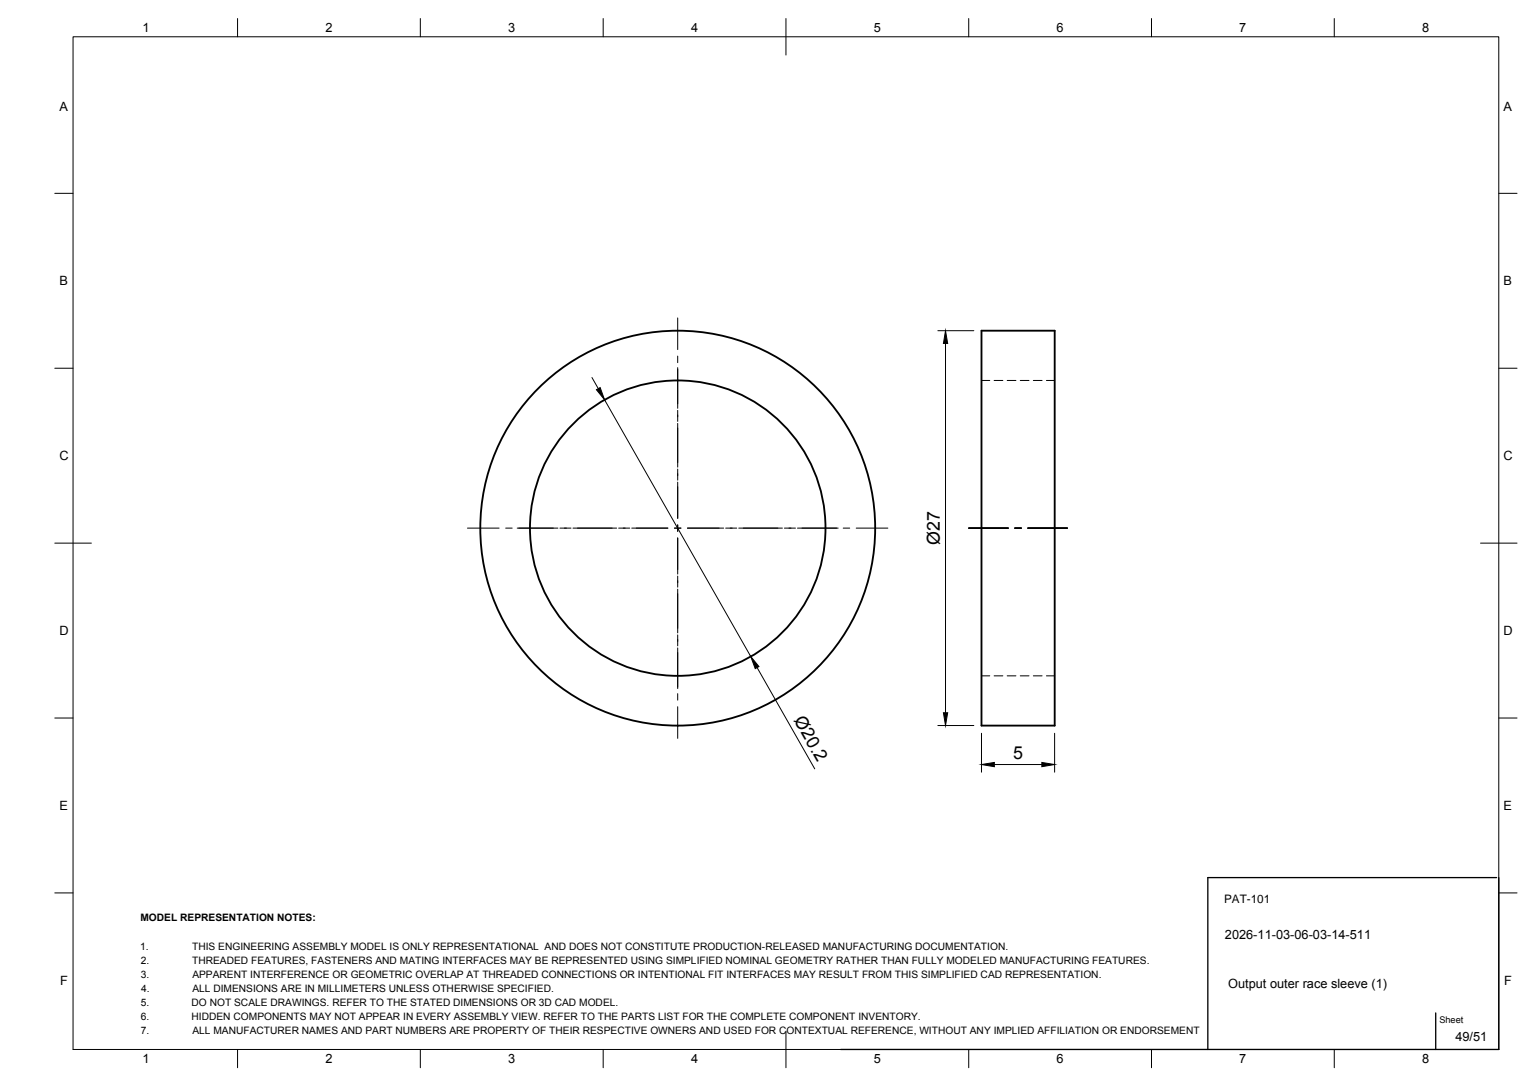
ISO-10303-21;
HEADER;
/* Generated by software containing ST-Developer
 * from STEP Tools, Inc. (www.steptools.com) 
 */

FILE_DESCRIPTION(
/* description */ ('Spur gear reduction stage 2-1 on bearing plates'),
/* implementation_level */ '2;1');

FILE_NAME(
/* name */ 'Output outer race sleeve (1).step',
/* time_stamp */ '2026-10-28T03:22:07-07:00',
/* author */ (''),
/* organization */ (''),
/* preprocessor_version */ 'ST-DEVELOPER v20.2',
/* originating_system */ 'Autodesk Translation Framework v15.17.0.0',
/* authorisation */ '');

FILE_SCHEMA (('AUTOMOTIVE_DESIGN { 1 0 10303 214 3 1 1 }'));
ENDSEC;

DATA;
#10=MECHANICAL_DESIGN_GEOMETRIC_PRESENTATION_REPRESENTATION('',(#1001),#53909);
#900=SHAPE_REPRESENTATION_RELATIONSHIP('SRR','None',#54131,#943);
#943=ADVANCED_BREP_SHAPE_REPRESENTATION('',(#1056),#53905);
#1001=STYLED_ITEM('',(#54397),#1056);
#1056=MANIFOLD_SOLID_BREP('Body1',#11328);
#1232=FACE_BOUND('',#2780,.T.);
#1233=FACE_BOUND('',#2782,.T.);
#1436=PLANE('',#12754);
#1437=PLANE('',#12755);
#1957=FACE_OUTER_BOUND('',#2777,.T.);
#1958=FACE_OUTER_BOUND('',#2778,.T.);
#1959=FACE_OUTER_BOUND('',#2779,.T.);
#1960=FACE_OUTER_BOUND('',#2781,.T.);
#2777=EDGE_LOOP('',(#9320,#9321,#9322,#9323));
#2778=EDGE_LOOP('',(#9324,#9325,#9326,#9327));
#2779=EDGE_LOOP('',(#9328));
#2780=EDGE_LOOP('',(#9329));
#2781=EDGE_LOOP('',(#9330));
#2782=EDGE_LOOP('',(#9331));
#3400=LINE('',#30116,#4041);
#3401=LINE('',#30122,#4042);
#4041=VECTOR('',#15293,1.01);
#4042=VECTOR('',#15300,1.35);
#4692=CIRCLE('',#12749,1.01);
#4693=CIRCLE('',#12750,1.01);
#4694=CIRCLE('',#12752,1.35);
#4695=CIRCLE('',#12753,1.35);
#5452=VERTEX_POINT('',#30113);
#5453=VERTEX_POINT('',#30115);
#5454=VERTEX_POINT('',#30119);
#5455=VERTEX_POINT('',#30121);
#6802=EDGE_CURVE('',#5452,#5452,#4692,.T.);
#6803=EDGE_CURVE('',#5452,#5453,#3400,.T.);
#6804=EDGE_CURVE('',#5453,#5453,#4693,.T.);
#6805=EDGE_CURVE('',#5454,#5454,#4694,.T.);
#6806=EDGE_CURVE('',#5454,#5455,#3401,.T.);
#6807=EDGE_CURVE('',#5455,#5455,#4695,.T.);
#9320=ORIENTED_EDGE('',*,*,#6802,.F.);
#9321=ORIENTED_EDGE('',*,*,#6803,.T.);
#9322=ORIENTED_EDGE('',*,*,#6804,.T.);
#9323=ORIENTED_EDGE('',*,*,#6803,.F.);
#9324=ORIENTED_EDGE('',*,*,#6805,.F.);
#9325=ORIENTED_EDGE('',*,*,#6806,.T.);
#9326=ORIENTED_EDGE('',*,*,#6807,.T.);
#9327=ORIENTED_EDGE('',*,*,#6806,.F.);
#9328=ORIENTED_EDGE('',*,*,#6805,.T.);
#9329=ORIENTED_EDGE('',*,*,#6802,.T.);
#9330=ORIENTED_EDGE('',*,*,#6807,.F.);
#9331=ORIENTED_EDGE('',*,*,#6804,.F.);
#10578=CYLINDRICAL_SURFACE('',#12748,1.01);
#10579=CYLINDRICAL_SURFACE('',#12751,1.35);
#11077=ADVANCED_FACE('',(#1957),#10578,.F.);
#11078=ADVANCED_FACE('',(#1958),#10579,.T.);
#11079=ADVANCED_FACE('',(#1959,#1232),#1436,.T.);
#11080=ADVANCED_FACE('',(#1960,#1233),#1437,.F.);
#11328=CLOSED_SHELL('',(#11077,#11078,#11079,#11080));
#12747=AXIS2_PLACEMENT_3D('',#30111,#15287,#15288);
#12748=AXIS2_PLACEMENT_3D('',#30112,#15289,#15290);
#12749=AXIS2_PLACEMENT_3D('',#30114,#15291,#15292);
#12750=AXIS2_PLACEMENT_3D('',#30117,#15294,#15295);
#12751=AXIS2_PLACEMENT_3D('',#30118,#15296,#15297);
#12752=AXIS2_PLACEMENT_3D('',#30120,#15298,#15299);
#12753=AXIS2_PLACEMENT_3D('',#30123,#15301,#15302);
#12754=AXIS2_PLACEMENT_3D('',#30124,#15303,#15304);
#12755=AXIS2_PLACEMENT_3D('',#30125,#15305,#15306);
#15287=DIRECTION('axis',(0.,0.,1.));
#15288=DIRECTION('refdir',(1.,0.,0.));
#15289=DIRECTION('center_axis',(0.,1.,0.));
#15290=DIRECTION('ref_axis',(1.,0.,0.));
#15291=DIRECTION('center_axis',(0.,-1.,0.));
#15292=DIRECTION('ref_axis',(1.,0.,0.));
#15293=DIRECTION('',(0.,-1.,0.));
#15294=DIRECTION('center_axis',(0.,-1.,0.));
#15295=DIRECTION('ref_axis',(1.,0.,0.));
#15296=DIRECTION('center_axis',(0.,1.,0.));
#15297=DIRECTION('ref_axis',(1.,0.,0.));
#15298=DIRECTION('center_axis',(0.,1.,0.));
#15299=DIRECTION('ref_axis',(1.,0.,0.));
#15300=DIRECTION('',(0.,-1.,0.));
#15301=DIRECTION('center_axis',(0.,1.,0.));
#15302=DIRECTION('ref_axis',(1.,0.,0.));
#15303=DIRECTION('center_axis',(0.,1.,0.));
#15304=DIRECTION('ref_axis',(1.,0.,0.));
#15305=DIRECTION('center_axis',(0.,1.,0.));
#15306=DIRECTION('ref_axis',(1.,0.,0.));
#30111=CARTESIAN_POINT('',(0.,0.,0.));
#30112=CARTESIAN_POINT('Origin',(0.,4.2,0.));
#30113=CARTESIAN_POINT('',(-1.01,4.7,1.23689326713883E-16));
#30114=CARTESIAN_POINT('Origin',(0.,4.7,0.));
#30115=CARTESIAN_POINT('',(-1.01,4.2,1.23689326713883E-16));
#30116=CARTESIAN_POINT('',(-1.01,4.2,1.23689326713883E-16));
#30117=CARTESIAN_POINT('Origin',(0.,4.2,0.));
#30118=CARTESIAN_POINT('Origin',(0.,4.2,0.));
#30119=CARTESIAN_POINT('',(-1.35,4.7,1.65327317884893E-16));
#30120=CARTESIAN_POINT('Origin',(0.,4.7,0.));
#30121=CARTESIAN_POINT('',(-1.35,4.2,1.65327317884893E-16));
#30122=CARTESIAN_POINT('',(-1.35,4.2,1.65327317884893E-16));
#30123=CARTESIAN_POINT('Origin',(0.,4.2,0.));
#30124=CARTESIAN_POINT('Origin',(0.,4.7,0.));
#30125=CARTESIAN_POINT('Origin',(0.,4.2,0.));
#53855=UNCERTAINTY_MEASURE_WITH_UNIT(LENGTH_MEASURE(0.001),#53910,
'DISTANCE_ACCURACY_VALUE',
'Maximum model space distance between geometric entities at asserted c
onnectivities');
#53859=UNCERTAINTY_MEASURE_WITH_UNIT(LENGTH_MEASURE(0.001),#53910,
'DISTANCE_ACCURACY_VALUE',
'Maximum model space distance between geometric entities at asserted c
onnectivities');
#53905=(
GEOMETRIC_REPRESENTATION_CONTEXT(3)
GLOBAL_UNCERTAINTY_ASSIGNED_CONTEXT((#53855))
GLOBAL_UNIT_ASSIGNED_CONTEXT((#53910,#53912,#53913))
REPRESENTATION_CONTEXT('','3D')
);
#53909=(
GEOMETRIC_REPRESENTATION_CONTEXT(3)
GLOBAL_UNCERTAINTY_ASSIGNED_CONTEXT((#53859))
GLOBAL_UNIT_ASSIGNED_CONTEXT((#53910,#53912,#53913))
REPRESENTATION_CONTEXT('','3D')
);
#53910=(
LENGTH_UNIT()
NAMED_UNIT(*)
SI_UNIT(.CENTI.,.METRE.)
);
#53912=(
NAMED_UNIT(*)
PLANE_ANGLE_UNIT()
SI_UNIT($,.RADIAN.)
);
#53913=(
NAMED_UNIT(*)
SI_UNIT($,.STERADIAN.)
SOLID_ANGLE_UNIT()
);
#53959=SHAPE_DEFINITION_REPRESENTATION(#54057,#54131);
#54057=PRODUCT_DEFINITION_SHAPE('',$,#54181);
#54131=SHAPE_REPRESENTATION('',(#12747),#53905);
#54135=PRODUCT_DEFINITION_CONTEXT('part definition',#54284,'design');
#54181=PRODUCT_DEFINITION('Output outer race sleeve (1)',
'Output outer race sleeve (1)',#54230,#54135);
#54230=PRODUCT_DEFINITION_FORMATION('',$,#54331);
#54284=APPLICATION_CONTEXT(
'Core Data for Automotive Mechanical Design Process');
#54285=PRODUCT_CONTEXT('part definition',#54284,'mechanical');
#54331=PRODUCT('Output outer race sleeve (1)',
'Output outer race sleeve (1)','Output outer race sleeve (1)',(#54285));
#54391=COLOUR_RGB('Grey',0.48,0.52,0.57);
#54392=FILL_AREA_STYLE_COLOUR('',#54391);
#54393=FILL_AREA_STYLE('',(#54392));
#54394=SURFACE_STYLE_FILL_AREA(#54393);
#54395=SURFACE_SIDE_STYLE('',(#54394));
#54396=SURFACE_STYLE_USAGE(.BOTH.,#54395);
#54397=PRESENTATION_STYLE_ASSIGNMENT((#54396));
ENDSEC;
END-ISO-10303-21;
